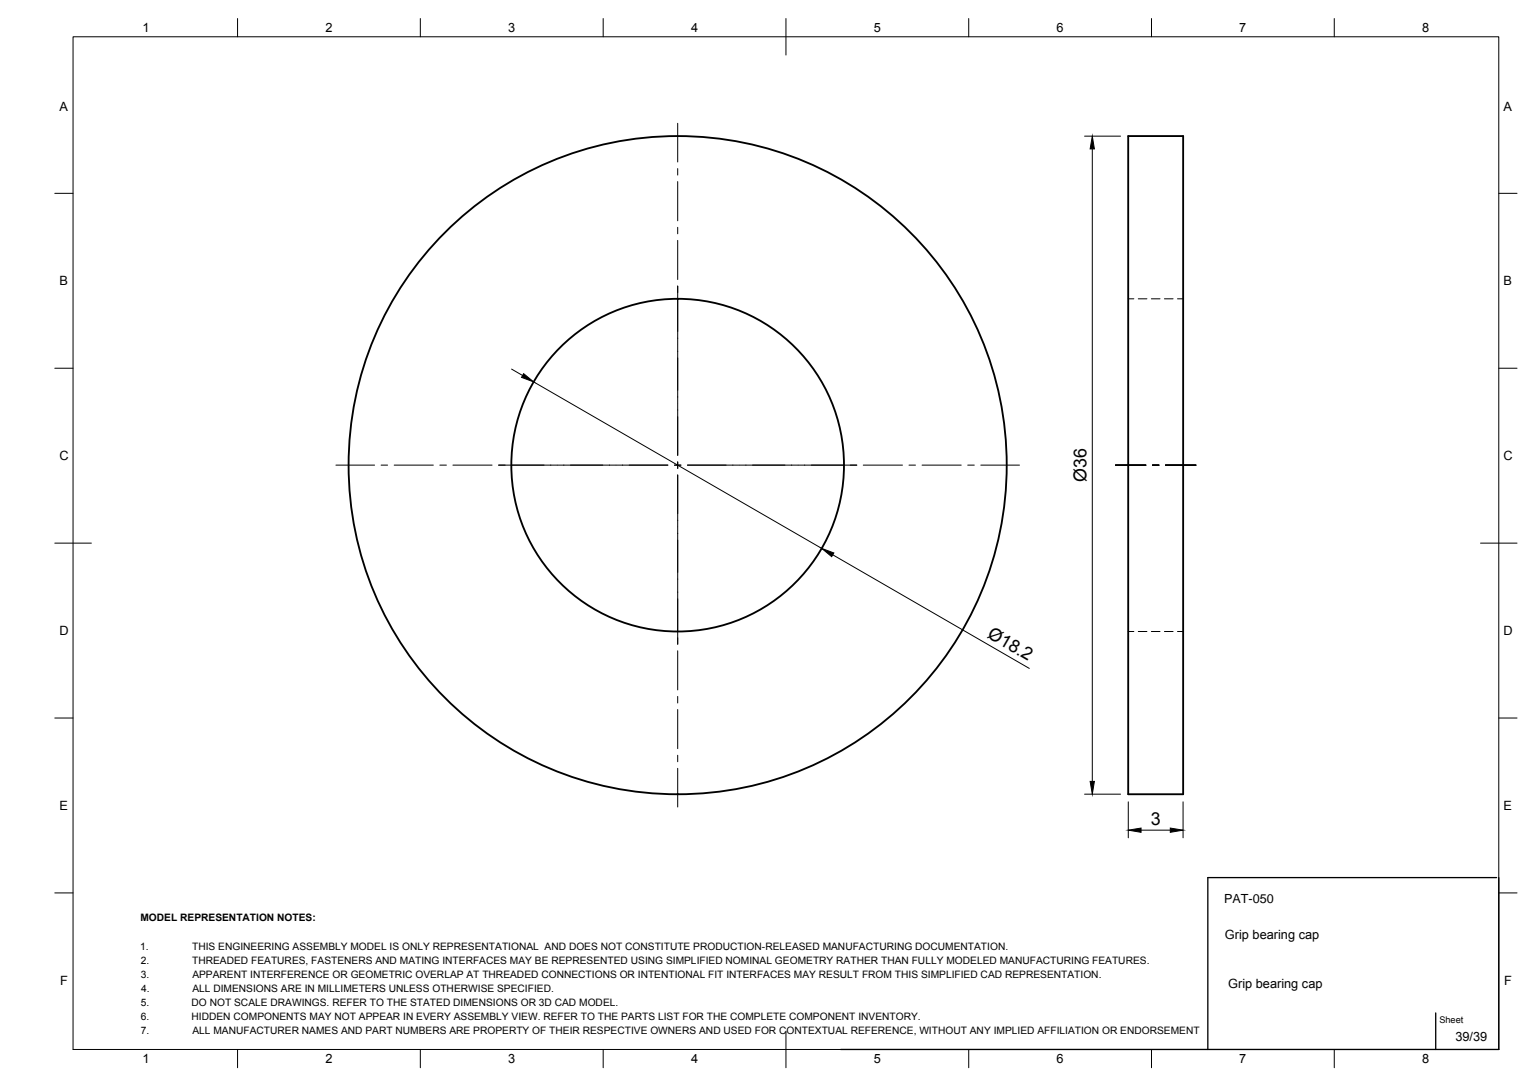
ISO-10303-21;
HEADER;
/* Generated by software containing ST-Developer
 * from STEP Tools, Inc. (www.steptools.com) 
 */

FILE_DESCRIPTION(
/* description */ ('Hand wheel with handle and shaft collar'),
/* implementation_level */ '2;1');

FILE_NAME(
/* name */ 'Grip bearing cap.step',
/* time_stamp */ '2026-10-28T03:23:19-07:00',
/* author */ (''),
/* organization */ (''),
/* preprocessor_version */ 'ST-DEVELOPER v20.2',
/* originating_system */ 'Autodesk Translation Framework v15.17.0.0',
/* authorisation */ '');

FILE_SCHEMA (('AUTOMOTIVE_DESIGN { 1 0 10303 214 3 1 1 }'));
ENDSEC;

DATA;
#10=MECHANICAL_DESIGN_GEOMETRIC_PRESENTATION_REPRESENTATION('',(#441),#10510);
#362=SHAPE_REPRESENTATION_RELATIONSHIP('SRR','None',#10682,#394);
#394=ADVANCED_BREP_SHAPE_REPRESENTATION('',(#485),#10509);
#441=STYLED_ITEM('',(#10908),#485);
#485=MANIFOLD_SOLID_BREP('Body1',#5343);
#596=FACE_BOUND('',#1510,.T.);
#597=FACE_BOUND('',#1512,.T.);
#761=PLANE('',#6412);
#762=PLANE('',#6413);
#1078=FACE_OUTER_BOUND('',#1507,.T.);
#1079=FACE_OUTER_BOUND('',#1508,.T.);
#1080=FACE_OUTER_BOUND('',#1509,.T.);
#1081=FACE_OUTER_BOUND('',#1511,.T.);
#1507=EDGE_LOOP('',(#4867,#4868,#4869,#4870));
#1508=EDGE_LOOP('',(#4871,#4872,#4873,#4874));
#1509=EDGE_LOOP('',(#4875));
#1510=EDGE_LOOP('',(#4876));
#1511=EDGE_LOOP('',(#4877));
#1512=EDGE_LOOP('',(#4878));
#1821=LINE('',#10418,#2131);
#1822=LINE('',#10424,#2132);
#2131=VECTOR('',#8149,0.91);
#2132=VECTOR('',#8156,1.8);
#2440=CIRCLE('',#6407,0.91);
#2441=CIRCLE('',#6408,0.91);
#2442=CIRCLE('',#6410,1.8);
#2443=CIRCLE('',#6411,1.8);
#2892=VERTEX_POINT('',#10415);
#2893=VERTEX_POINT('',#10417);
#2894=VERTEX_POINT('',#10421);
#2895=VERTEX_POINT('',#10423);
#3551=EDGE_CURVE('',#2892,#2892,#2440,.T.);
#3552=EDGE_CURVE('',#2892,#2893,#1821,.T.);
#3553=EDGE_CURVE('',#2893,#2893,#2441,.T.);
#3554=EDGE_CURVE('',#2894,#2894,#2442,.T.);
#3555=EDGE_CURVE('',#2894,#2895,#1822,.T.);
#3556=EDGE_CURVE('',#2895,#2895,#2443,.T.);
#4867=ORIENTED_EDGE('',*,*,#3551,.F.);
#4868=ORIENTED_EDGE('',*,*,#3552,.T.);
#4869=ORIENTED_EDGE('',*,*,#3553,.T.);
#4870=ORIENTED_EDGE('',*,*,#3552,.F.);
#4871=ORIENTED_EDGE('',*,*,#3554,.F.);
#4872=ORIENTED_EDGE('',*,*,#3555,.T.);
#4873=ORIENTED_EDGE('',*,*,#3556,.T.);
#4874=ORIENTED_EDGE('',*,*,#3555,.F.);
#4875=ORIENTED_EDGE('',*,*,#3554,.T.);
#4876=ORIENTED_EDGE('',*,*,#3551,.T.);
#4877=ORIENTED_EDGE('',*,*,#3556,.F.);
#4878=ORIENTED_EDGE('',*,*,#3553,.F.);
#4973=CYLINDRICAL_SURFACE('',#6406,0.91);
#4974=CYLINDRICAL_SURFACE('',#6409,1.8);
#5290=ADVANCED_FACE('',(#1078),#4973,.F.);
#5291=ADVANCED_FACE('',(#1079),#4974,.T.);
#5292=ADVANCED_FACE('',(#1080,#596),#761,.T.);
#5293=ADVANCED_FACE('',(#1081,#597),#762,.F.);
#5343=CLOSED_SHELL('',(#5290,#5291,#5292,#5293));
#6405=AXIS2_PLACEMENT_3D('',#10413,#8143,#8144);
#6406=AXIS2_PLACEMENT_3D('',#10414,#8145,#8146);
#6407=AXIS2_PLACEMENT_3D('',#10416,#8147,#8148);
#6408=AXIS2_PLACEMENT_3D('',#10419,#8150,#8151);
#6409=AXIS2_PLACEMENT_3D('',#10420,#8152,#8153);
#6410=AXIS2_PLACEMENT_3D('',#10422,#8154,#8155);
#6411=AXIS2_PLACEMENT_3D('',#10425,#8157,#8158);
#6412=AXIS2_PLACEMENT_3D('',#10426,#8159,#8160);
#6413=AXIS2_PLACEMENT_3D('',#10427,#8161,#8162);
#8143=DIRECTION('axis',(0.,0.,1.));
#8144=DIRECTION('refdir',(1.,0.,0.));
#8145=DIRECTION('center_axis',(0.,1.,0.));
#8146=DIRECTION('ref_axis',(1.,0.,0.));
#8147=DIRECTION('center_axis',(0.,-1.,0.));
#8148=DIRECTION('ref_axis',(1.,0.,0.));
#8149=DIRECTION('',(0.,-1.,0.));
#8150=DIRECTION('center_axis',(0.,-1.,0.));
#8151=DIRECTION('ref_axis',(1.,0.,0.));
#8152=DIRECTION('center_axis',(0.,1.,0.));
#8153=DIRECTION('ref_axis',(1.,0.,0.));
#8154=DIRECTION('center_axis',(0.,1.,0.));
#8155=DIRECTION('ref_axis',(1.,0.,0.));
#8156=DIRECTION('',(0.,-1.,0.));
#8157=DIRECTION('center_axis',(0.,1.,0.));
#8158=DIRECTION('ref_axis',(1.,0.,0.));
#8159=DIRECTION('center_axis',(0.,1.,0.));
#8160=DIRECTION('ref_axis',(1.,0.,0.));
#8161=DIRECTION('center_axis',(0.,1.,0.));
#8162=DIRECTION('ref_axis',(1.,0.,0.));
#10413=CARTESIAN_POINT('',(0.,0.,0.));
#10414=CARTESIAN_POINT('Origin',(6.5,-4.55,10.));
#10415=CARTESIAN_POINT('',(5.59,-4.25,10.));
#10416=CARTESIAN_POINT('Origin',(6.5,-4.25,10.));
#10417=CARTESIAN_POINT('',(5.59,-4.55,10.));
#10418=CARTESIAN_POINT('',(5.59,-4.55,10.));
#10419=CARTESIAN_POINT('Origin',(6.5,-4.55,10.));
#10420=CARTESIAN_POINT('Origin',(6.5,-4.55,10.));
#10421=CARTESIAN_POINT('',(4.7,-4.25,10.));
#10422=CARTESIAN_POINT('Origin',(6.5,-4.25,10.));
#10423=CARTESIAN_POINT('',(4.7,-4.55,10.));
#10424=CARTESIAN_POINT('',(4.7,-4.55,10.));
#10425=CARTESIAN_POINT('Origin',(6.5,-4.55,10.));
#10426=CARTESIAN_POINT('Origin',(6.5,-4.25,10.));
#10427=CARTESIAN_POINT('Origin',(6.5,-4.55,10.));
#10470=UNCERTAINTY_MEASURE_WITH_UNIT(LENGTH_MEASURE(0.001),#10511,
'DISTANCE_ACCURACY_VALUE',
'Maximum model space distance between geometric entities at asserted c
onnectivities');
#10471=UNCERTAINTY_MEASURE_WITH_UNIT(LENGTH_MEASURE(0.001),#10511,
'DISTANCE_ACCURACY_VALUE',
'Maximum model space distance between geometric entities at asserted c
onnectivities');
#10509=(
GEOMETRIC_REPRESENTATION_CONTEXT(3)
GLOBAL_UNCERTAINTY_ASSIGNED_CONTEXT((#10470))
GLOBAL_UNIT_ASSIGNED_CONTEXT((#10511,#10513,#10514))
REPRESENTATION_CONTEXT('','3D')
);
#10510=(
GEOMETRIC_REPRESENTATION_CONTEXT(3)
GLOBAL_UNCERTAINTY_ASSIGNED_CONTEXT((#10471))
GLOBAL_UNIT_ASSIGNED_CONTEXT((#10511,#10513,#10514))
REPRESENTATION_CONTEXT('','3D')
);
#10511=(
LENGTH_UNIT()
NAMED_UNIT(*)
SI_UNIT(.CENTI.,.METRE.)
);
#10513=(
NAMED_UNIT(*)
PLANE_ANGLE_UNIT()
SI_UNIT($,.RADIAN.)
);
#10514=(
NAMED_UNIT(*)
SI_UNIT($,.STERADIAN.)
SOLID_ANGLE_UNIT()
);
#10552=SHAPE_DEFINITION_REPRESENTATION(#10639,#10682);
#10639=PRODUCT_DEFINITION_SHAPE('',$,#10721);
#10682=SHAPE_REPRESENTATION('',(#6405),#10509);
#10683=PRODUCT_DEFINITION_CONTEXT('part definition',#10799,'design');
#10721=PRODUCT_DEFINITION('Grip bearing cap','Grip bearing cap',#10759,
#10683);
#10759=PRODUCT_DEFINITION_FORMATION('',$,#10838);
#10799=APPLICATION_CONTEXT(
'Core Data for Automotive Mechanical Design Process');
#10800=PRODUCT_CONTEXT('part definition',#10799,'mechanical');
#10838=PRODUCT('Grip bearing cap','Grip bearing cap','Grip bearing cap',
(#10800));
#10902=COLOUR_RGB('Grey',0.48,0.52,0.57);
#10903=FILL_AREA_STYLE_COLOUR('',#10902);
#10904=FILL_AREA_STYLE('',(#10903));
#10905=SURFACE_STYLE_FILL_AREA(#10904);
#10906=SURFACE_SIDE_STYLE('',(#10905));
#10907=SURFACE_STYLE_USAGE(.BOTH.,#10906);
#10908=PRESENTATION_STYLE_ASSIGNMENT((#10907));
ENDSEC;
END-ISO-10303-21;
